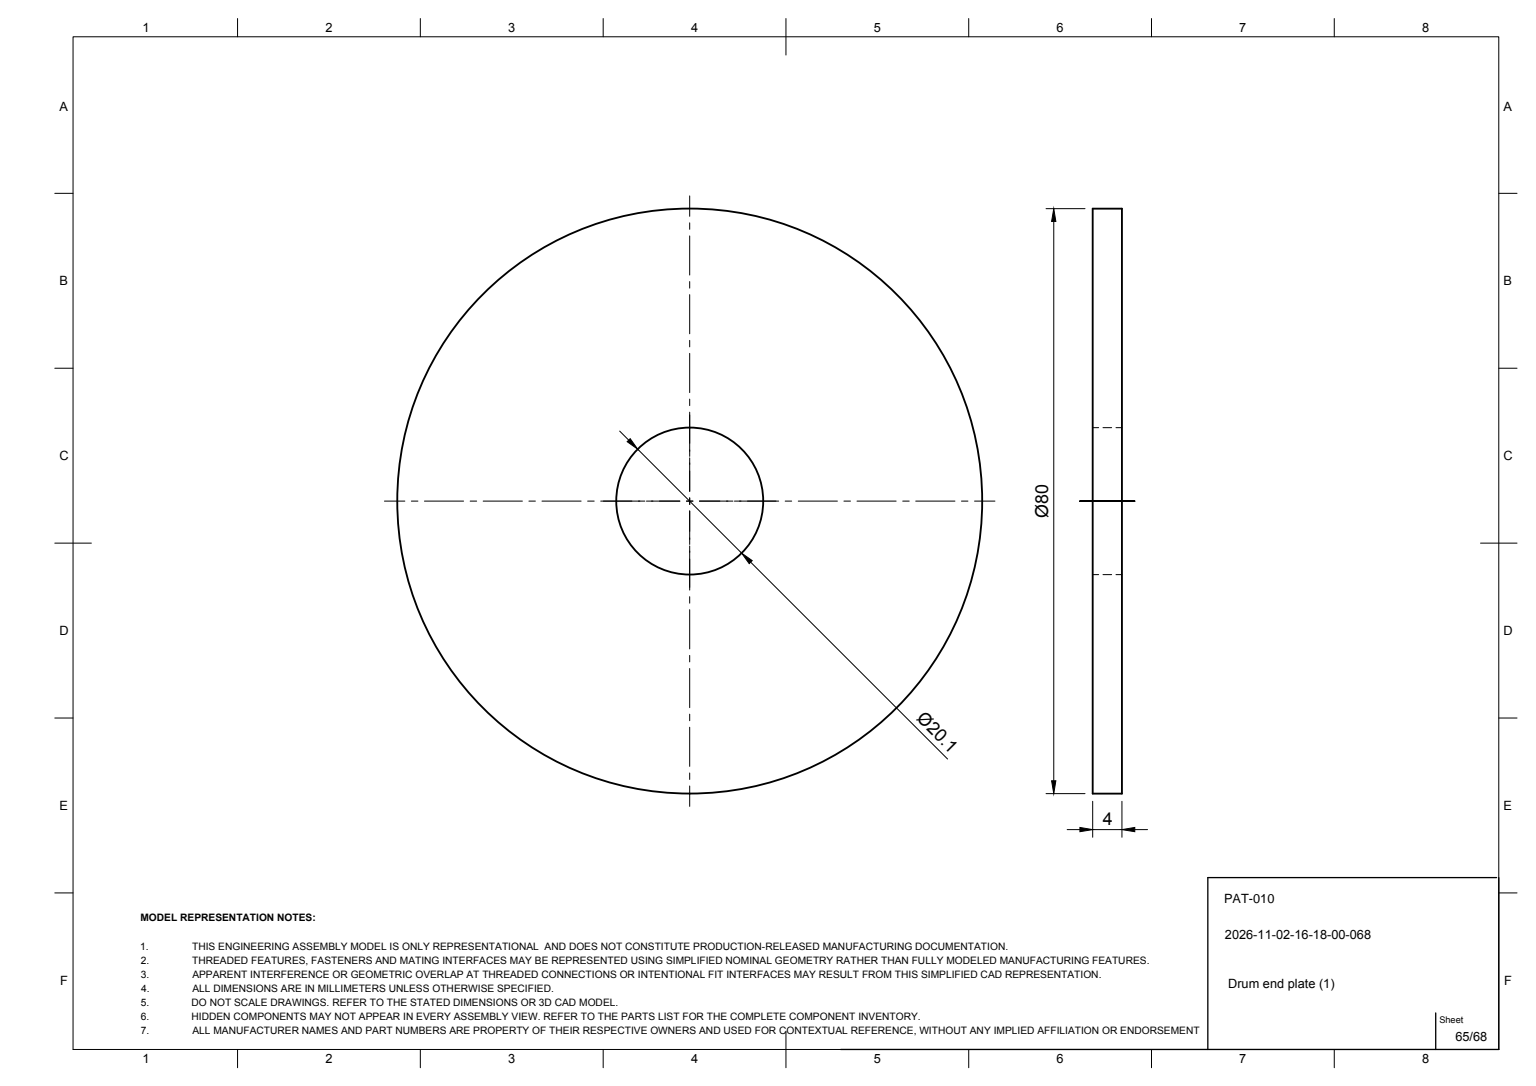
ISO-10303-21;
HEADER;
/* Generated by software containing ST-Developer
 * from STEP Tools, Inc. (www.steptools.com) 
 */

FILE_DESCRIPTION(
/* description */ ('Belt conveyor head drive unit'),
/* implementation_level */ '2;1');

FILE_NAME(
/* name */ 'Drum end plate (1).step',
/* time_stamp */ '2026-10-28T03:26:19-07:00',
/* author */ (''),
/* organization */ (''),
/* preprocessor_version */ 'ST-DEVELOPER v20.2',
/* originating_system */ 'Autodesk Translation Framework v15.17.0.0',
/* authorisation */ '');

FILE_SCHEMA (('AUTOMOTIVE_DESIGN { 1 0 10303 214 3 1 1 }'));
ENDSEC;

DATA;
#10=MECHANICAL_DESIGN_GEOMETRIC_PRESENTATION_REPRESENTATION('',(#926),#27069);
#772=SHAPE_REPRESENTATION_RELATIONSHIP('SRR','None',#27421,#841);
#841=ADVANCED_BREP_SHAPE_REPRESENTATION('',(#1007),#27063);
#926=STYLED_ITEM('',(#27790),#1007);
#1007=MANIFOLD_SOLID_BREP('Body1',#13795);
#1254=FACE_BOUND('',#3338,.T.);
#1255=FACE_BOUND('',#3340,.T.);
#1598=PLANE('',#15984);
#1599=PLANE('',#15985);
#2293=FACE_OUTER_BOUND('',#3335,.T.);
#2294=FACE_OUTER_BOUND('',#3336,.T.);
#2295=FACE_OUTER_BOUND('',#3337,.T.);
#2296=FACE_OUTER_BOUND('',#3339,.T.);
#3335=EDGE_LOOP('',(#11782,#11783,#11784,#11785));
#3336=EDGE_LOOP('',(#11786,#11787,#11788,#11789));
#3337=EDGE_LOOP('',(#11790));
#3338=EDGE_LOOP('',(#11791));
#3339=EDGE_LOOP('',(#11792));
#3340=EDGE_LOOP('',(#11793));
#4143=LINE('',#25637,#4935);
#4144=LINE('',#25643,#4936);
#4935=VECTOR('',#19915,1.005);
#4936=VECTOR('',#19922,4.);
#5755=CIRCLE('',#15979,1.005);
#5756=CIRCLE('',#15980,1.005);
#5757=CIRCLE('',#15982,4.);
#5758=CIRCLE('',#15983,4.);
#6919=VERTEX_POINT('',#25634);
#6920=VERTEX_POINT('',#25636);
#6921=VERTEX_POINT('',#25640);
#6922=VERTEX_POINT('',#25642);
#8583=EDGE_CURVE('',#6919,#6919,#5755,.T.);
#8584=EDGE_CURVE('',#6919,#6920,#4143,.T.);
#8585=EDGE_CURVE('',#6920,#6920,#5756,.T.);
#8586=EDGE_CURVE('',#6921,#6921,#5757,.T.);
#8587=EDGE_CURVE('',#6921,#6922,#4144,.T.);
#8588=EDGE_CURVE('',#6922,#6922,#5758,.T.);
#11782=ORIENTED_EDGE('',*,*,#8583,.F.);
#11783=ORIENTED_EDGE('',*,*,#8584,.T.);
#11784=ORIENTED_EDGE('',*,*,#8585,.T.);
#11785=ORIENTED_EDGE('',*,*,#8584,.F.);
#11786=ORIENTED_EDGE('',*,*,#8586,.F.);
#11787=ORIENTED_EDGE('',*,*,#8587,.T.);
#11788=ORIENTED_EDGE('',*,*,#8588,.T.);
#11789=ORIENTED_EDGE('',*,*,#8587,.F.);
#11790=ORIENTED_EDGE('',*,*,#8586,.T.);
#11791=ORIENTED_EDGE('',*,*,#8583,.T.);
#11792=ORIENTED_EDGE('',*,*,#8588,.F.);
#11793=ORIENTED_EDGE('',*,*,#8585,.F.);
#12813=CYLINDRICAL_SURFACE('',#15978,1.005);
#12814=CYLINDRICAL_SURFACE('',#15981,4.);
#13572=ADVANCED_FACE('',(#2293),#12813,.F.);
#13573=ADVANCED_FACE('',(#2294),#12814,.T.);
#13574=ADVANCED_FACE('',(#2295,#1254),#1598,.T.);
#13575=ADVANCED_FACE('',(#2296,#1255),#1599,.F.);
#13795=CLOSED_SHELL('',(#13572,#13573,#13574,#13575));
#15977=AXIS2_PLACEMENT_3D('',#25632,#19909,#19910);
#15978=AXIS2_PLACEMENT_3D('',#25633,#19911,#19912);
#15979=AXIS2_PLACEMENT_3D('',#25635,#19913,#19914);
#15980=AXIS2_PLACEMENT_3D('',#25638,#19916,#19917);
#15981=AXIS2_PLACEMENT_3D('',#25639,#19918,#19919);
#15982=AXIS2_PLACEMENT_3D('',#25641,#19920,#19921);
#15983=AXIS2_PLACEMENT_3D('',#25644,#19923,#19924);
#15984=AXIS2_PLACEMENT_3D('',#25645,#19925,#19926);
#15985=AXIS2_PLACEMENT_3D('',#25646,#19927,#19928);
#19909=DIRECTION('axis',(0.,0.,1.));
#19910=DIRECTION('refdir',(1.,0.,0.));
#19911=DIRECTION('center_axis',(0.,1.,0.));
#19912=DIRECTION('ref_axis',(1.,0.,0.));
#19913=DIRECTION('center_axis',(0.,-1.,0.));
#19914=DIRECTION('ref_axis',(1.,0.,0.));
#19915=DIRECTION('',(0.,-1.,0.));
#19916=DIRECTION('center_axis',(0.,-1.,0.));
#19917=DIRECTION('ref_axis',(1.,0.,0.));
#19918=DIRECTION('center_axis',(0.,1.,0.));
#19919=DIRECTION('ref_axis',(1.,0.,0.));
#19920=DIRECTION('center_axis',(0.,1.,0.));
#19921=DIRECTION('ref_axis',(1.,0.,0.));
#19922=DIRECTION('',(0.,-1.,0.));
#19923=DIRECTION('center_axis',(0.,1.,0.));
#19924=DIRECTION('ref_axis',(1.,0.,0.));
#19925=DIRECTION('center_axis',(0.,1.,0.));
#19926=DIRECTION('ref_axis',(1.,0.,0.));
#19927=DIRECTION('center_axis',(0.,1.,0.));
#19928=DIRECTION('ref_axis',(1.,0.,0.));
#25632=CARTESIAN_POINT('',(0.,0.,0.));
#25633=CARTESIAN_POINT('Origin',(6.97091003018116,37.,7.));
#25634=CARTESIAN_POINT('',(5.96591003018116,37.4,7.));
#25635=CARTESIAN_POINT('Origin',(6.97091003018116,37.4,7.));
#25636=CARTESIAN_POINT('',(5.96591003018116,37.,7.));
#25637=CARTESIAN_POINT('',(5.96591003018116,37.,7.));
#25638=CARTESIAN_POINT('Origin',(6.97091003018116,37.,7.));
#25639=CARTESIAN_POINT('Origin',(6.97091003018116,37.,7.));
#25640=CARTESIAN_POINT('',(2.97091003018116,37.4,7.));
#25641=CARTESIAN_POINT('Origin',(6.97091003018116,37.4,7.));
#25642=CARTESIAN_POINT('',(2.97091003018116,37.,7.));
#25643=CARTESIAN_POINT('',(2.97091003018116,37.,7.));
#25644=CARTESIAN_POINT('Origin',(6.97091003018116,37.,7.));
#25645=CARTESIAN_POINT('Origin',(6.97091003018116,37.4,7.));
#25646=CARTESIAN_POINT('Origin',(6.97091003018116,37.,7.));
#26986=UNCERTAINTY_MEASURE_WITH_UNIT(LENGTH_MEASURE(0.001),#27070,
'DISTANCE_ACCURACY_VALUE',
'Maximum model space distance between geometric entities at asserted c
onnectivities');
#26992=UNCERTAINTY_MEASURE_WITH_UNIT(LENGTH_MEASURE(0.001),#27070,
'DISTANCE_ACCURACY_VALUE',
'Maximum model space distance between geometric entities at asserted c
onnectivities');
#27063=(
GEOMETRIC_REPRESENTATION_CONTEXT(3)
GLOBAL_UNCERTAINTY_ASSIGNED_CONTEXT((#26986))
GLOBAL_UNIT_ASSIGNED_CONTEXT((#27070,#27072,#27073))
REPRESENTATION_CONTEXT('','3D')
);
#27069=(
GEOMETRIC_REPRESENTATION_CONTEXT(3)
GLOBAL_UNCERTAINTY_ASSIGNED_CONTEXT((#26992))
GLOBAL_UNIT_ASSIGNED_CONTEXT((#27070,#27072,#27073))
REPRESENTATION_CONTEXT('','3D')
);
#27070=(
LENGTH_UNIT()
NAMED_UNIT(*)
SI_UNIT(.CENTI.,.METRE.)
);
#27072=(
NAMED_UNIT(*)
PLANE_ANGLE_UNIT()
SI_UNIT($,.RADIAN.)
);
#27073=(
NAMED_UNIT(*)
SI_UNIT($,.STERADIAN.)
SOLID_ANGLE_UNIT()
);
#27144=SHAPE_DEFINITION_REPRESENTATION(#27232,#27421);
#27232=PRODUCT_DEFINITION_SHAPE('',$,#27498);
#27421=SHAPE_REPRESENTATION('',(#15977),#27063);
#27427=PRODUCT_DEFINITION_CONTEXT('part definition',#27657,'design');
#27498=PRODUCT_DEFINITION('Drum end plate (1)','Drum end plate (1)',#27574,
#27427);
#27574=PRODUCT_DEFINITION_FORMATION('',$,#27729);
#27657=APPLICATION_CONTEXT(
'Core Data for Automotive Mechanical Design Process');
#27658=PRODUCT_CONTEXT('part definition',#27657,'mechanical');
#27729=PRODUCT('Drum end plate (1)','Drum end plate (1)','Drum end plate (1)',
(#27658));
#27784=COLOUR_RGB('Sky Blue',0.24,0.69,0.87);
#27785=FILL_AREA_STYLE_COLOUR('',#27784);
#27786=FILL_AREA_STYLE('',(#27785));
#27787=SURFACE_STYLE_FILL_AREA(#27786);
#27788=SURFACE_SIDE_STYLE('',(#27787));
#27789=SURFACE_STYLE_USAGE(.BOTH.,#27788);
#27790=PRESENTATION_STYLE_ASSIGNMENT((#27789));
ENDSEC;
END-ISO-10303-21;
